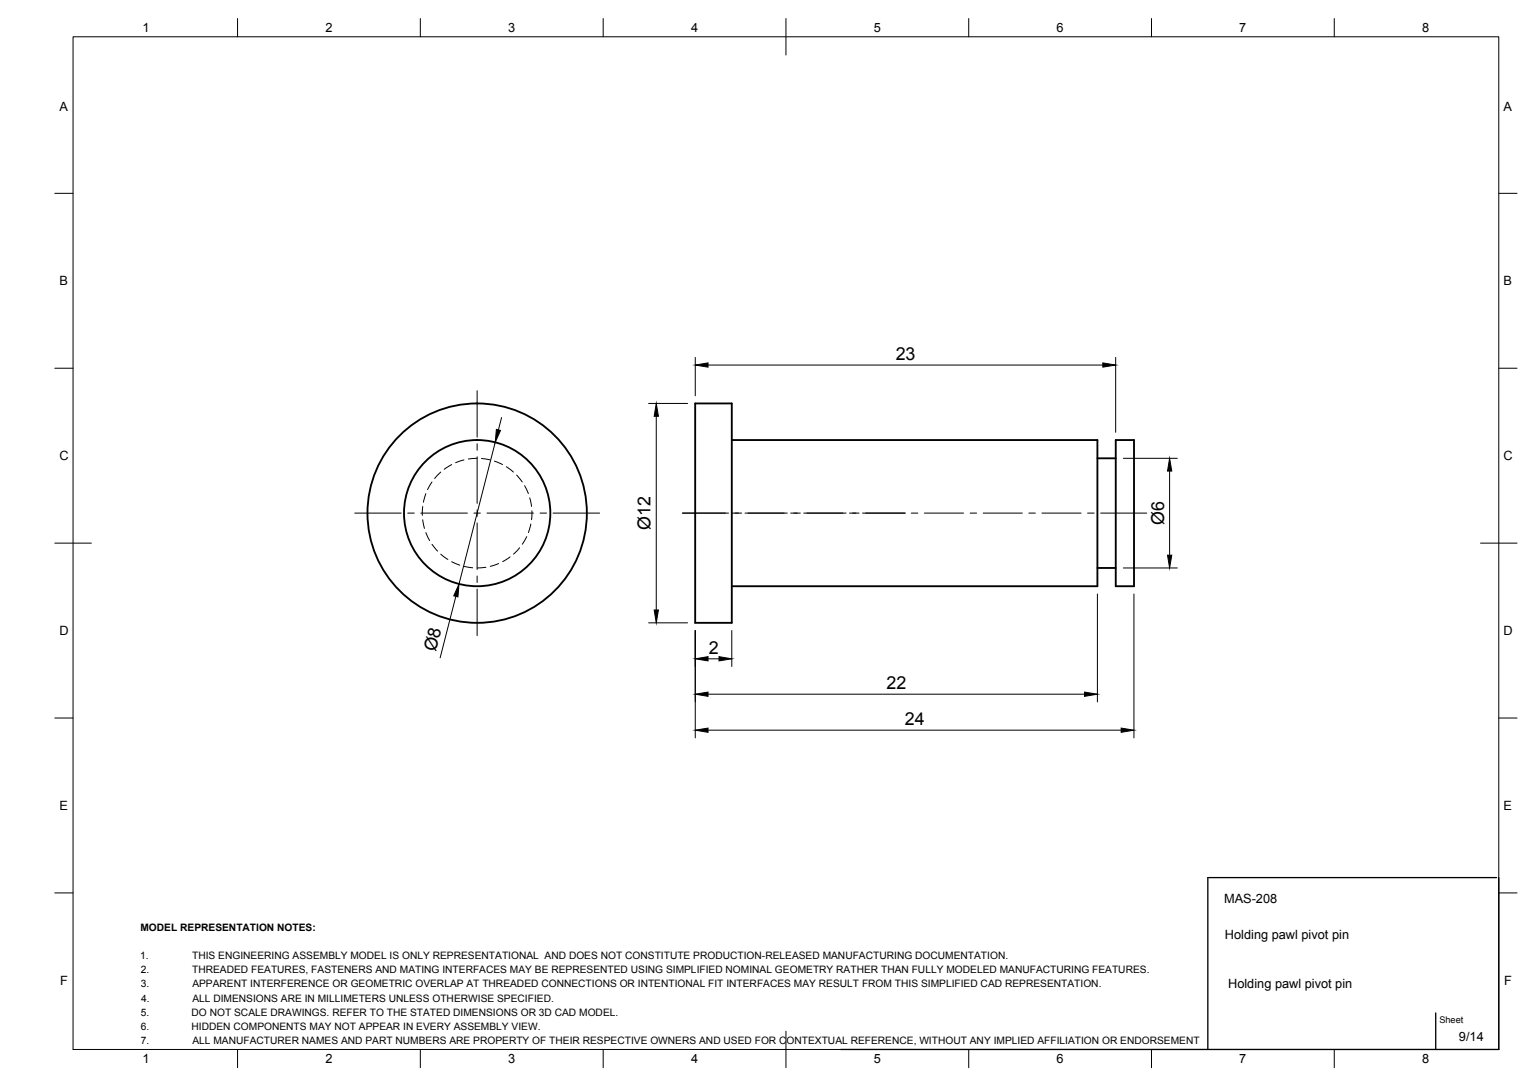
ISO-10303-21;
HEADER;
/* Generated by software containing ST-Developer
 * from STEP Tools, Inc. (www.steptools.com) 
 */

FILE_DESCRIPTION(
/* description */ ('Independent vertical20-tooth ratchet advance with repeated integral-c
ounterweight gravity pawls, swinging drive lever, bronze sleeves and f
ully retained axle stacks.18degpertooth. Native revolutes; geometric c
ycle checking rather than automatic contact/rolling dynamics. Gravity 
closing checked from actual pawl center of mass. Backplate/foot suppor
ts unit. Fits, torque, holding force, wear and life unassigned.'),
/* implementation_level */ '2;1');

FILE_NAME(
/* name */ 'Holding pawl pivot pin.step',
/* time_stamp */ '2026-11-09T06:25:53-08:00',
/* author */ (''),
/* organization */ (''),
/* preprocessor_version */ 'ST-DEVELOPER v20.2',
/* originating_system */ 'Autodesk Translation Framework v15.17.0.0',
/* authorisation */ '');

FILE_SCHEMA (('AUTOMOTIVE_DESIGN { 1 0 10303 214 3 1 1 }'));
ENDSEC;

DATA;
#10=MECHANICAL_DESIGN_GEOMETRIC_PRESENTATION_REPRESENTATION('',(#128),#4643);
#100=SHAPE_REPRESENTATION_RELATIONSHIP('SRR','None',#4705,#114);
#114=ADVANCED_BREP_SHAPE_REPRESENTATION('',(#142),#4634);
#128=STYLED_ITEM('',(#4782),#142);
#142=MANIFOLD_SOLID_BREP('Body1',#2664);
#177=FACE_BOUND('',#571,.T.);
#178=FACE_BOUND('',#573,.T.);
#179=FACE_BOUND('',#576,.T.);
#264=PLANE('',#2964);
#265=PLANE('',#2966);
#266=PLANE('',#2970);
#267=PLANE('',#2975);
#268=PLANE('',#2977);
#394=FACE_OUTER_BOUND('',#569,.T.);
#395=FACE_OUTER_BOUND('',#570,.T.);
#396=FACE_OUTER_BOUND('',#572,.T.);
#397=FACE_OUTER_BOUND('',#574,.T.);
#398=FACE_OUTER_BOUND('',#575,.T.);
#399=FACE_OUTER_BOUND('',#577,.T.);
#400=FACE_OUTER_BOUND('',#578,.T.);
#401=FACE_OUTER_BOUND('',#579,.T.);
#402=FACE_OUTER_BOUND('',#580,.T.);
#569=EDGE_LOOP('',(#2245,#2246,#2247,#2248));
#570=EDGE_LOOP('',(#2249));
#571=EDGE_LOOP('',(#2250));
#572=EDGE_LOOP('',(#2251));
#573=EDGE_LOOP('',(#2252));
#574=EDGE_LOOP('',(#2253,#2254,#2255,#2256));
#575=EDGE_LOOP('',(#2257));
#576=EDGE_LOOP('',(#2258));
#577=EDGE_LOOP('',(#2259,#2260,#2261,#2262));
#578=EDGE_LOOP('',(#2263));
#579=EDGE_LOOP('',(#2264,#2265,#2266,#2267));
#580=EDGE_LOOP('',(#2268));
#829=LINE('',#4338,#1091);
#830=LINE('',#4349,#1092);
#831=LINE('',#4357,#1093);
#832=LINE('',#4361,#1094);
#1091=VECTOR('',#3543,3.);
#1092=VECTOR('',#3558,4.);
#1093=VECTOR('',#3567,6.);
#1094=VECTOR('',#3574,4.);
#1203=CIRCLE('',#2962,3.);
#1204=CIRCLE('',#2963,3.);
#1205=CIRCLE('',#2965,4.);
#1206=CIRCLE('',#2967,4.);
#1207=CIRCLE('',#2969,4.);
#1208=CIRCLE('',#2971,6.);
#1209=CIRCLE('',#2972,4.);
#1210=CIRCLE('',#2974,6.);
#1389=VERTEX_POINT('',#4335);
#1390=VERTEX_POINT('',#4337);
#1391=VERTEX_POINT('',#4341);
#1392=VERTEX_POINT('',#4344);
#1393=VERTEX_POINT('',#4347);
#1394=VERTEX_POINT('',#4351);
#1395=VERTEX_POINT('',#4353);
#1396=VERTEX_POINT('',#4356);
#1687=EDGE_CURVE('',#1389,#1389,#1203,.T.);
#1688=EDGE_CURVE('',#1389,#1390,#829,.T.);
#1689=EDGE_CURVE('',#1390,#1390,#1204,.T.);
#1690=EDGE_CURVE('',#1391,#1391,#1205,.T.);
#1691=EDGE_CURVE('',#1392,#1392,#1206,.T.);
#1692=EDGE_CURVE('',#1393,#1393,#1207,.T.);
#1693=EDGE_CURVE('',#1393,#1392,#830,.T.);
#1694=EDGE_CURVE('',#1394,#1394,#1208,.T.);
#1695=EDGE_CURVE('',#1395,#1395,#1209,.T.);
#1696=EDGE_CURVE('',#1394,#1396,#831,.T.);
#1697=EDGE_CURVE('',#1396,#1396,#1210,.T.);
#1698=EDGE_CURVE('',#1391,#1395,#832,.T.);
#2245=ORIENTED_EDGE('',*,*,#1687,.T.);
#2246=ORIENTED_EDGE('',*,*,#1688,.T.);
#2247=ORIENTED_EDGE('',*,*,#1689,.F.);
#2248=ORIENTED_EDGE('',*,*,#1688,.F.);
#2249=ORIENTED_EDGE('',*,*,#1690,.F.);
#2250=ORIENTED_EDGE('',*,*,#1687,.F.);
#2251=ORIENTED_EDGE('',*,*,#1691,.F.);
#2252=ORIENTED_EDGE('',*,*,#1689,.T.);
#2253=ORIENTED_EDGE('',*,*,#1692,.F.);
#2254=ORIENTED_EDGE('',*,*,#1693,.T.);
#2255=ORIENTED_EDGE('',*,*,#1691,.T.);
#2256=ORIENTED_EDGE('',*,*,#1693,.F.);
#2257=ORIENTED_EDGE('',*,*,#1694,.T.);
#2258=ORIENTED_EDGE('',*,*,#1695,.F.);
#2259=ORIENTED_EDGE('',*,*,#1694,.F.);
#2260=ORIENTED_EDGE('',*,*,#1696,.T.);
#2261=ORIENTED_EDGE('',*,*,#1697,.T.);
#2262=ORIENTED_EDGE('',*,*,#1696,.F.);
#2263=ORIENTED_EDGE('',*,*,#1697,.F.);
#2264=ORIENTED_EDGE('',*,*,#1690,.T.);
#2265=ORIENTED_EDGE('',*,*,#1698,.T.);
#2266=ORIENTED_EDGE('',*,*,#1695,.T.);
#2267=ORIENTED_EDGE('',*,*,#1698,.F.);
#2268=ORIENTED_EDGE('',*,*,#1692,.T.);
#2491=CYLINDRICAL_SURFACE('',#2961,3.);
#2492=CYLINDRICAL_SURFACE('',#2968,4.);
#2493=CYLINDRICAL_SURFACE('',#2973,6.);
#2494=CYLINDRICAL_SURFACE('',#2976,4.);
#2600=ADVANCED_FACE('',(#394),#2491,.T.);
#2601=ADVANCED_FACE('',(#395,#177),#264,.F.);
#2602=ADVANCED_FACE('',(#396,#178),#265,.F.);
#2603=ADVANCED_FACE('',(#397),#2492,.T.);
#2604=ADVANCED_FACE('',(#398,#179),#266,.T.);
#2605=ADVANCED_FACE('',(#399),#2493,.T.);
#2606=ADVANCED_FACE('',(#400),#267,.F.);
#2607=ADVANCED_FACE('',(#401),#2494,.T.);
#2608=ADVANCED_FACE('',(#402),#268,.T.);
#2664=CLOSED_SHELL('',(#2600,#2601,#2602,#2603,#2604,#2605,#2606,#2607,
#2608));
#2960=AXIS2_PLACEMENT_3D('',#4333,#3537,#3538);
#2961=AXIS2_PLACEMENT_3D('',#4334,#3539,#3540);
#2962=AXIS2_PLACEMENT_3D('',#4336,#3541,#3542);
#2963=AXIS2_PLACEMENT_3D('',#4339,#3544,#3545);
#2964=AXIS2_PLACEMENT_3D('',#4340,#3546,#3547);
#2965=AXIS2_PLACEMENT_3D('',#4342,#3548,#3549);
#2966=AXIS2_PLACEMENT_3D('',#4343,#3550,#3551);
#2967=AXIS2_PLACEMENT_3D('',#4345,#3552,#3553);
#2968=AXIS2_PLACEMENT_3D('',#4346,#3554,#3555);
#2969=AXIS2_PLACEMENT_3D('',#4348,#3556,#3557);
#2970=AXIS2_PLACEMENT_3D('',#4350,#3559,#3560);
#2971=AXIS2_PLACEMENT_3D('',#4352,#3561,#3562);
#2972=AXIS2_PLACEMENT_3D('',#4354,#3563,#3564);
#2973=AXIS2_PLACEMENT_3D('',#4355,#3565,#3566);
#2974=AXIS2_PLACEMENT_3D('',#4358,#3568,#3569);
#2975=AXIS2_PLACEMENT_3D('',#4359,#3570,#3571);
#2976=AXIS2_PLACEMENT_3D('',#4360,#3572,#3573);
#2977=AXIS2_PLACEMENT_3D('',#4362,#3575,#3576);
#3537=DIRECTION('axis',(0.,0.,1.));
#3538=DIRECTION('refdir',(1.,0.,0.));
#3539=DIRECTION('center_axis',(0.,0.,1.));
#3540=DIRECTION('ref_axis',(1.,0.,0.));
#3541=DIRECTION('center_axis',(0.,0.,1.));
#3542=DIRECTION('ref_axis',(1.,0.,0.));
#3543=DIRECTION('',(0.,0.,1.));
#3544=DIRECTION('center_axis',(0.,0.,1.));
#3545=DIRECTION('ref_axis',(1.,0.,0.));
#3546=DIRECTION('center_axis',(0.,0.,-1.));
#3547=DIRECTION('ref_axis',(-1.,0.,0.));
#3548=DIRECTION('center_axis',(0.,0.,-1.));
#3549=DIRECTION('ref_axis',(1.,0.,0.));
#3550=DIRECTION('center_axis',(0.,0.,1.));
#3551=DIRECTION('ref_axis',(1.,0.,0.));
#3552=DIRECTION('center_axis',(0.,0.,1.));
#3553=DIRECTION('ref_axis',(1.,0.,0.));
#3554=DIRECTION('center_axis',(0.,0.,1.));
#3555=DIRECTION('ref_axis',(1.,0.,0.));
#3556=DIRECTION('center_axis',(0.,0.,1.));
#3557=DIRECTION('ref_axis',(1.,0.,0.));
#3558=DIRECTION('',(0.,0.,-1.));
#3559=DIRECTION('center_axis',(0.,0.,1.));
#3560=DIRECTION('ref_axis',(1.,0.,0.));
#3561=DIRECTION('center_axis',(0.,0.,1.));
#3562=DIRECTION('ref_axis',(1.,0.,0.));
#3563=DIRECTION('center_axis',(0.,0.,1.));
#3564=DIRECTION('ref_axis',(1.,0.,0.));
#3565=DIRECTION('center_axis',(0.,0.,1.));
#3566=DIRECTION('ref_axis',(1.,0.,0.));
#3567=DIRECTION('',(0.,0.,-1.));
#3568=DIRECTION('center_axis',(0.,0.,1.));
#3569=DIRECTION('ref_axis',(1.,0.,0.));
#3570=DIRECTION('center_axis',(0.,0.,1.));
#3571=DIRECTION('ref_axis',(1.,0.,0.));
#3572=DIRECTION('center_axis',(0.,0.,1.));
#3573=DIRECTION('ref_axis',(1.,0.,0.));
#3574=DIRECTION('',(0.,0.,-1.));
#3575=DIRECTION('center_axis',(0.,0.,1.));
#3576=DIRECTION('ref_axis',(1.,0.,0.));
#4333=CARTESIAN_POINT('',(0.,0.,0.));
#4334=CARTESIAN_POINT('Origin',(0.,0.,20.5));
#4335=CARTESIAN_POINT('',(-3.,-3.67394039744206E-16,20.));
#4336=CARTESIAN_POINT('Origin',(0.,0.,20.));
#4337=CARTESIAN_POINT('',(-3.,-3.67394039744206E-16,21.));
#4338=CARTESIAN_POINT('',(-3.,-3.67394039744206E-16,20.5));
#4339=CARTESIAN_POINT('Origin',(0.,0.,21.));
#4340=CARTESIAN_POINT('Origin',(7.,0.,20.));
#4341=CARTESIAN_POINT('',(-4.,4.89858719658941E-16,20.));
#4342=CARTESIAN_POINT('Origin',(0.,0.,20.));
#4343=CARTESIAN_POINT('Origin',(3.,0.,21.));
#4344=CARTESIAN_POINT('',(-4.,-4.89858719658941E-16,21.));
#4345=CARTESIAN_POINT('Origin',(0.,0.,21.));
#4346=CARTESIAN_POINT('Origin',(0.,0.,0.));
#4347=CARTESIAN_POINT('',(-4.,-4.89858719658941E-16,22.));
#4348=CARTESIAN_POINT('Origin',(0.,0.,22.));
#4349=CARTESIAN_POINT('',(-4.,-4.89858719658941E-16,0.));
#4350=CARTESIAN_POINT('Origin',(0.,0.,0.));
#4351=CARTESIAN_POINT('',(-6.,-7.34788079488412E-16,0.));
#4352=CARTESIAN_POINT('Origin',(0.,0.,0.));
#4353=CARTESIAN_POINT('',(-4.,-4.89858719658941E-16,0.));
#4354=CARTESIAN_POINT('Origin',(0.,0.,0.));
#4355=CARTESIAN_POINT('Origin',(0.,0.,-2.));
#4356=CARTESIAN_POINT('',(-6.,-7.34788079488412E-16,-2.));
#4357=CARTESIAN_POINT('',(-6.,-7.34788079488412E-16,-2.));
#4358=CARTESIAN_POINT('Origin',(0.,0.,-2.));
#4359=CARTESIAN_POINT('Origin',(0.,0.,-2.));
#4360=CARTESIAN_POINT('Origin',(0.,0.,0.));
#4361=CARTESIAN_POINT('',(-4.,-4.89858719658941E-16,0.));
#4362=CARTESIAN_POINT('Origin',(0.,0.,22.));
#4618=UNCERTAINTY_MEASURE_WITH_UNIT(LENGTH_MEASURE(0.01),#4644,
'DISTANCE_ACCURACY_VALUE',
'Maximum model space distance between geometric entities at asserted c
onnectivities');
#4627=UNCERTAINTY_MEASURE_WITH_UNIT(LENGTH_MEASURE(0.01),#4644,
'DISTANCE_ACCURACY_VALUE',
'Maximum model space distance between geometric entities at asserted c
onnectivities');
#4634=(
GEOMETRIC_REPRESENTATION_CONTEXT(3)
GLOBAL_UNCERTAINTY_ASSIGNED_CONTEXT((#4618))
GLOBAL_UNIT_ASSIGNED_CONTEXT((#4644,#4646,#4647))
REPRESENTATION_CONTEXT('','3D')
);
#4643=(
GEOMETRIC_REPRESENTATION_CONTEXT(3)
GLOBAL_UNCERTAINTY_ASSIGNED_CONTEXT((#4627))
GLOBAL_UNIT_ASSIGNED_CONTEXT((#4644,#4646,#4647))
REPRESENTATION_CONTEXT('','3D')
);
#4644=(
LENGTH_UNIT()
NAMED_UNIT(*)
SI_UNIT(.MILLI.,.METRE.)
);
#4646=(
NAMED_UNIT(*)
PLANE_ANGLE_UNIT()
SI_UNIT($,.RADIAN.)
);
#4647=(
NAMED_UNIT(*)
SI_UNIT($,.STERADIAN.)
SOLID_ANGLE_UNIT()
);
#4654=SHAPE_DEFINITION_REPRESENTATION(#4669,#4705);
#4669=PRODUCT_DEFINITION_SHAPE('',$,#4721);
#4705=SHAPE_REPRESENTATION('',(#2960),#4634);
#4714=PRODUCT_DEFINITION_CONTEXT('part definition',#4761,'design');
#4721=PRODUCT_DEFINITION('Holding pawl pivot pin',
'Holding pawl pivot pin',#4736,#4714);
#4736=PRODUCT_DEFINITION_FORMATION('',$,#4769);
#4761=APPLICATION_CONTEXT(
'Core Data for Automotive Mechanical Design Process');
#4762=PRODUCT_CONTEXT('part definition',#4761,'mechanical');
#4769=PRODUCT('Holding pawl pivot pin','Holding pawl pivot pin',$,(#4762));
#4782=PRESENTATION_STYLE_ASSIGNMENT((#4791));
#4791=SURFACE_STYLE_USAGE(.BOTH.,#4800);
#4800=SURFACE_SIDE_STYLE('',(#4809));
#4809=SURFACE_STYLE_FILL_AREA(#4818);
#4818=FILL_AREA_STYLE('Axle gray',(#4827));
#4827=FILL_AREA_STYLE_COLOUR('Axle gray',#4836);
#4836=COLOUR_RGB('Axle gray',0.576470588235294,0.615686274509804,0.666666666666667);
ENDSEC;
END-ISO-10303-21;
